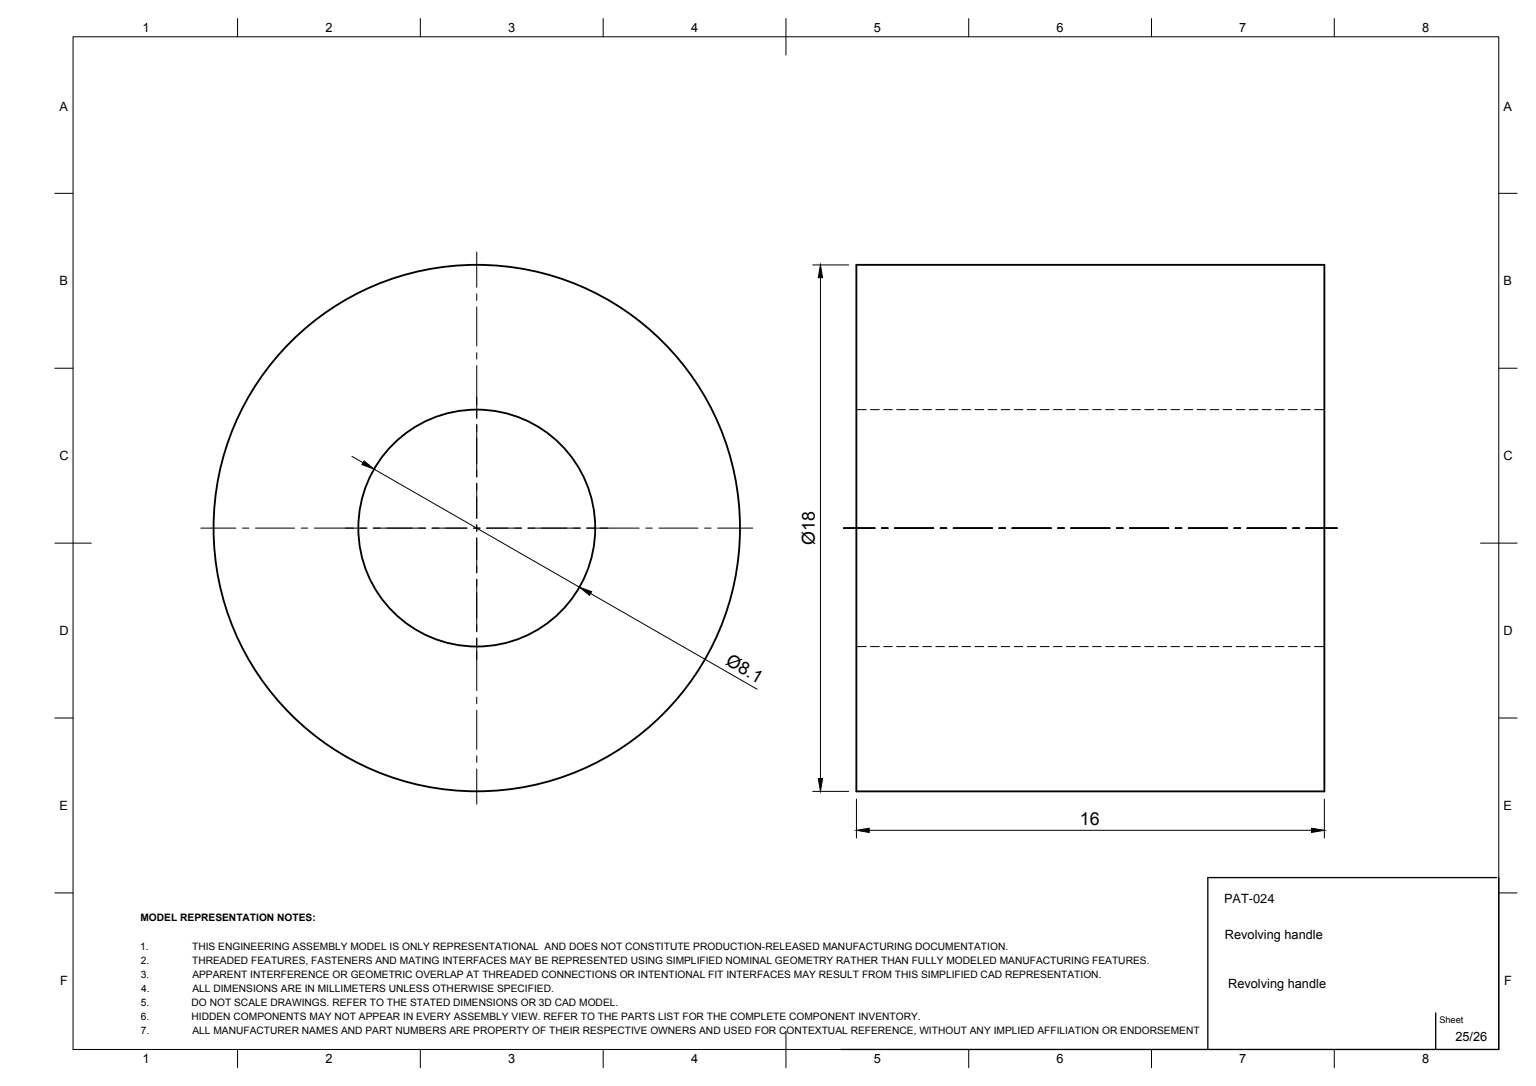
ISO-10303-21;
HEADER;
/* Generated by software containing ST-Developer
 * from STEP Tools, Inc. (www.steptools.com) 
 */

FILE_DESCRIPTION(
/* description */ ('Compact handwheel screw vise'),
/* implementation_level */ '2;1');

FILE_NAME(
/* name */ 'Revolving handle.step',
/* time_stamp */ '2026-10-29T16:08:22-07:00',
/* author */ (''),
/* organization */ (''),
/* preprocessor_version */ 'ST-DEVELOPER v20.2',
/* originating_system */ 'Autodesk Translation Framework v15.17.0.0',
/* authorisation */ '');

FILE_SCHEMA (('AUTOMOTIVE_DESIGN { 1 0 10303 214 3 1 1 }'));
ENDSEC;

DATA;
#10=MECHANICAL_DESIGN_GEOMETRIC_PRESENTATION_REPRESENTATION('',(#675),#25074);
#611=SHAPE_REPRESENTATION_RELATIONSHIP('SRR','None',#25222,#639);
#639=ADVANCED_BREP_SHAPE_REPRESENTATION('',(#708),#25069);
#675=STYLED_ITEM('',(#25432),#708);
#708=MANIFOLD_SOLID_BREP('Body1',#8086);
#816=FACE_BOUND('',#2012,.T.);
#817=FACE_BOUND('',#2014,.T.);
#978=PLANE('',#9106);
#979=PLANE('',#9107);
#1435=FACE_OUTER_BOUND('',#2009,.T.);
#1436=FACE_OUTER_BOUND('',#2010,.T.);
#1437=FACE_OUTER_BOUND('',#2011,.T.);
#1438=FACE_OUTER_BOUND('',#2013,.T.);
#2009=EDGE_LOOP('',(#7159,#7160,#7161,#7162));
#2010=EDGE_LOOP('',(#7163,#7164,#7165,#7166));
#2011=EDGE_LOOP('',(#7167));
#2012=EDGE_LOOP('',(#7168));
#2013=EDGE_LOOP('',(#7169));
#2014=EDGE_LOOP('',(#7170));
#2497=LINE('',#24774,#3005);
#2498=LINE('',#24780,#3006);
#3005=VECTOR('',#11041,0.405);
#3006=VECTOR('',#11048,0.9);
#3313=CIRCLE('',#9101,0.405);
#3314=CIRCLE('',#9102,0.405);
#3315=CIRCLE('',#9104,0.9);
#3316=CIRCLE('',#9105,0.9);
#4006=VERTEX_POINT('',#24771);
#4007=VERTEX_POINT('',#24773);
#4008=VERTEX_POINT('',#24777);
#4009=VERTEX_POINT('',#24779);
#5066=EDGE_CURVE('',#4006,#4006,#3313,.T.);
#5067=EDGE_CURVE('',#4006,#4007,#2497,.T.);
#5068=EDGE_CURVE('',#4007,#4007,#3314,.T.);
#5069=EDGE_CURVE('',#4008,#4008,#3315,.T.);
#5070=EDGE_CURVE('',#4008,#4009,#2498,.T.);
#5071=EDGE_CURVE('',#4009,#4009,#3316,.T.);
#7159=ORIENTED_EDGE('',*,*,#5066,.F.);
#7160=ORIENTED_EDGE('',*,*,#5067,.T.);
#7161=ORIENTED_EDGE('',*,*,#5068,.T.);
#7162=ORIENTED_EDGE('',*,*,#5067,.F.);
#7163=ORIENTED_EDGE('',*,*,#5069,.F.);
#7164=ORIENTED_EDGE('',*,*,#5070,.T.);
#7165=ORIENTED_EDGE('',*,*,#5071,.T.);
#7166=ORIENTED_EDGE('',*,*,#5070,.F.);
#7167=ORIENTED_EDGE('',*,*,#5069,.T.);
#7168=ORIENTED_EDGE('',*,*,#5066,.T.);
#7169=ORIENTED_EDGE('',*,*,#5071,.F.);
#7170=ORIENTED_EDGE('',*,*,#5068,.F.);
#7575=CYLINDRICAL_SURFACE('',#9100,0.405);
#7576=CYLINDRICAL_SURFACE('',#9103,0.9);
#8005=ADVANCED_FACE('',(#1435),#7575,.F.);
#8006=ADVANCED_FACE('',(#1436),#7576,.T.);
#8007=ADVANCED_FACE('',(#1437,#816),#978,.T.);
#8008=ADVANCED_FACE('',(#1438,#817),#979,.F.);
#8086=CLOSED_SHELL('',(#8005,#8006,#8007,#8008));
#9099=AXIS2_PLACEMENT_3D('',#24769,#11035,#11036);
#9100=AXIS2_PLACEMENT_3D('',#24770,#11037,#11038);
#9101=AXIS2_PLACEMENT_3D('',#24772,#11039,#11040);
#9102=AXIS2_PLACEMENT_3D('',#24775,#11042,#11043);
#9103=AXIS2_PLACEMENT_3D('',#24776,#11044,#11045);
#9104=AXIS2_PLACEMENT_3D('',#24778,#11046,#11047);
#9105=AXIS2_PLACEMENT_3D('',#24781,#11049,#11050);
#9106=AXIS2_PLACEMENT_3D('',#24782,#11051,#11052);
#9107=AXIS2_PLACEMENT_3D('',#24783,#11053,#11054);
#11035=DIRECTION('axis',(0.,0.,1.));
#11036=DIRECTION('refdir',(1.,0.,0.));
#11037=DIRECTION('center_axis',(1.,0.,0.));
#11038=DIRECTION('ref_axis',(0.,0.,-1.));
#11039=DIRECTION('center_axis',(-1.,0.,0.));
#11040=DIRECTION('ref_axis',(0.,0.,-1.));
#11041=DIRECTION('',(-1.,0.,0.));
#11042=DIRECTION('center_axis',(-1.,0.,0.));
#11043=DIRECTION('ref_axis',(0.,0.,-1.));
#11044=DIRECTION('center_axis',(1.,0.,0.));
#11045=DIRECTION('ref_axis',(0.,0.,-1.));
#11046=DIRECTION('center_axis',(1.,0.,0.));
#11047=DIRECTION('ref_axis',(0.,0.,-1.));
#11048=DIRECTION('',(-1.,0.,0.));
#11049=DIRECTION('center_axis',(1.,0.,0.));
#11050=DIRECTION('ref_axis',(0.,0.,-1.));
#11051=DIRECTION('center_axis',(1.,0.,0.));
#11052=DIRECTION('ref_axis',(0.,0.,-1.));
#11053=DIRECTION('center_axis',(1.,0.,0.));
#11054=DIRECTION('ref_axis',(0.,0.,-1.));
#24769=CARTESIAN_POINT('',(0.,0.,0.));
#24770=CARTESIAN_POINT('Origin',(29.4,0.,6.5));
#24771=CARTESIAN_POINT('',(31.,-4.95981953654678E-17,6.905));
#24772=CARTESIAN_POINT('Origin',(31.,0.,6.5));
#24773=CARTESIAN_POINT('',(29.4,-4.95981953654678E-17,6.905));
#24774=CARTESIAN_POINT('',(29.4,-4.95981953654678E-17,6.905));
#24775=CARTESIAN_POINT('Origin',(29.4,0.,6.5));
#24776=CARTESIAN_POINT('Origin',(29.4,0.,6.5));
#24777=CARTESIAN_POINT('',(31.,-1.10218211923262E-16,7.4));
#24778=CARTESIAN_POINT('Origin',(31.,0.,6.5));
#24779=CARTESIAN_POINT('',(29.4,-1.10218211923262E-16,7.4));
#24780=CARTESIAN_POINT('',(29.4,-1.10218211923262E-16,7.4));
#24781=CARTESIAN_POINT('Origin',(29.4,0.,6.5));
#24782=CARTESIAN_POINT('Origin',(31.,0.,6.5));
#24783=CARTESIAN_POINT('Origin',(29.4,0.,6.5));
#25035=UNCERTAINTY_MEASURE_WITH_UNIT(LENGTH_MEASURE(0.001),#25075,
'DISTANCE_ACCURACY_VALUE',
'Maximum model space distance between geometric entities at asserted c
onnectivities');
#25040=UNCERTAINTY_MEASURE_WITH_UNIT(LENGTH_MEASURE(0.001),#25075,
'DISTANCE_ACCURACY_VALUE',
'Maximum model space distance between geometric entities at asserted c
onnectivities');
#25069=(
GEOMETRIC_REPRESENTATION_CONTEXT(3)
GLOBAL_UNCERTAINTY_ASSIGNED_CONTEXT((#25035))
GLOBAL_UNIT_ASSIGNED_CONTEXT((#25075,#25077,#25078))
REPRESENTATION_CONTEXT('','3D')
);
#25074=(
GEOMETRIC_REPRESENTATION_CONTEXT(3)
GLOBAL_UNCERTAINTY_ASSIGNED_CONTEXT((#25040))
GLOBAL_UNIT_ASSIGNED_CONTEXT((#25075,#25077,#25078))
REPRESENTATION_CONTEXT('','3D')
);
#25075=(
LENGTH_UNIT()
NAMED_UNIT(*)
SI_UNIT(.CENTI.,.METRE.)
);
#25077=(
NAMED_UNIT(*)
PLANE_ANGLE_UNIT()
SI_UNIT($,.RADIAN.)
);
#25078=(
NAMED_UNIT(*)
SI_UNIT($,.STERADIAN.)
SOLID_ANGLE_UNIT()
);
#25107=SHAPE_DEFINITION_REPRESENTATION(#25156,#25222);
#25156=PRODUCT_DEFINITION_SHAPE('',$,#25256);
#25222=SHAPE_REPRESENTATION('',(#9099),#25069);
#25227=PRODUCT_DEFINITION_CONTEXT('part definition',#25328,'design');
#25256=PRODUCT_DEFINITION('Revolving handle','Revolving handle',#25289,
#25227);
#25289=PRODUCT_DEFINITION_FORMATION('',$,#25358);
#25328=APPLICATION_CONTEXT(
'Core Data for Automotive Mechanical Design Process');
#25329=PRODUCT_CONTEXT('part definition',#25328,'mechanical');
#25358=PRODUCT('Revolving handle','Revolving handle','Revolving handle',
(#25329));
#25426=COLOUR_RGB('Sky Blue',0.24,0.69,0.87);
#25427=FILL_AREA_STYLE_COLOUR('',#25426);
#25428=FILL_AREA_STYLE('',(#25427));
#25429=SURFACE_STYLE_FILL_AREA(#25428);
#25430=SURFACE_SIDE_STYLE('',(#25429));
#25431=SURFACE_STYLE_USAGE(.BOTH.,#25430);
#25432=PRESENTATION_STYLE_ASSIGNMENT((#25431));
ENDSEC;
END-ISO-10303-21;
